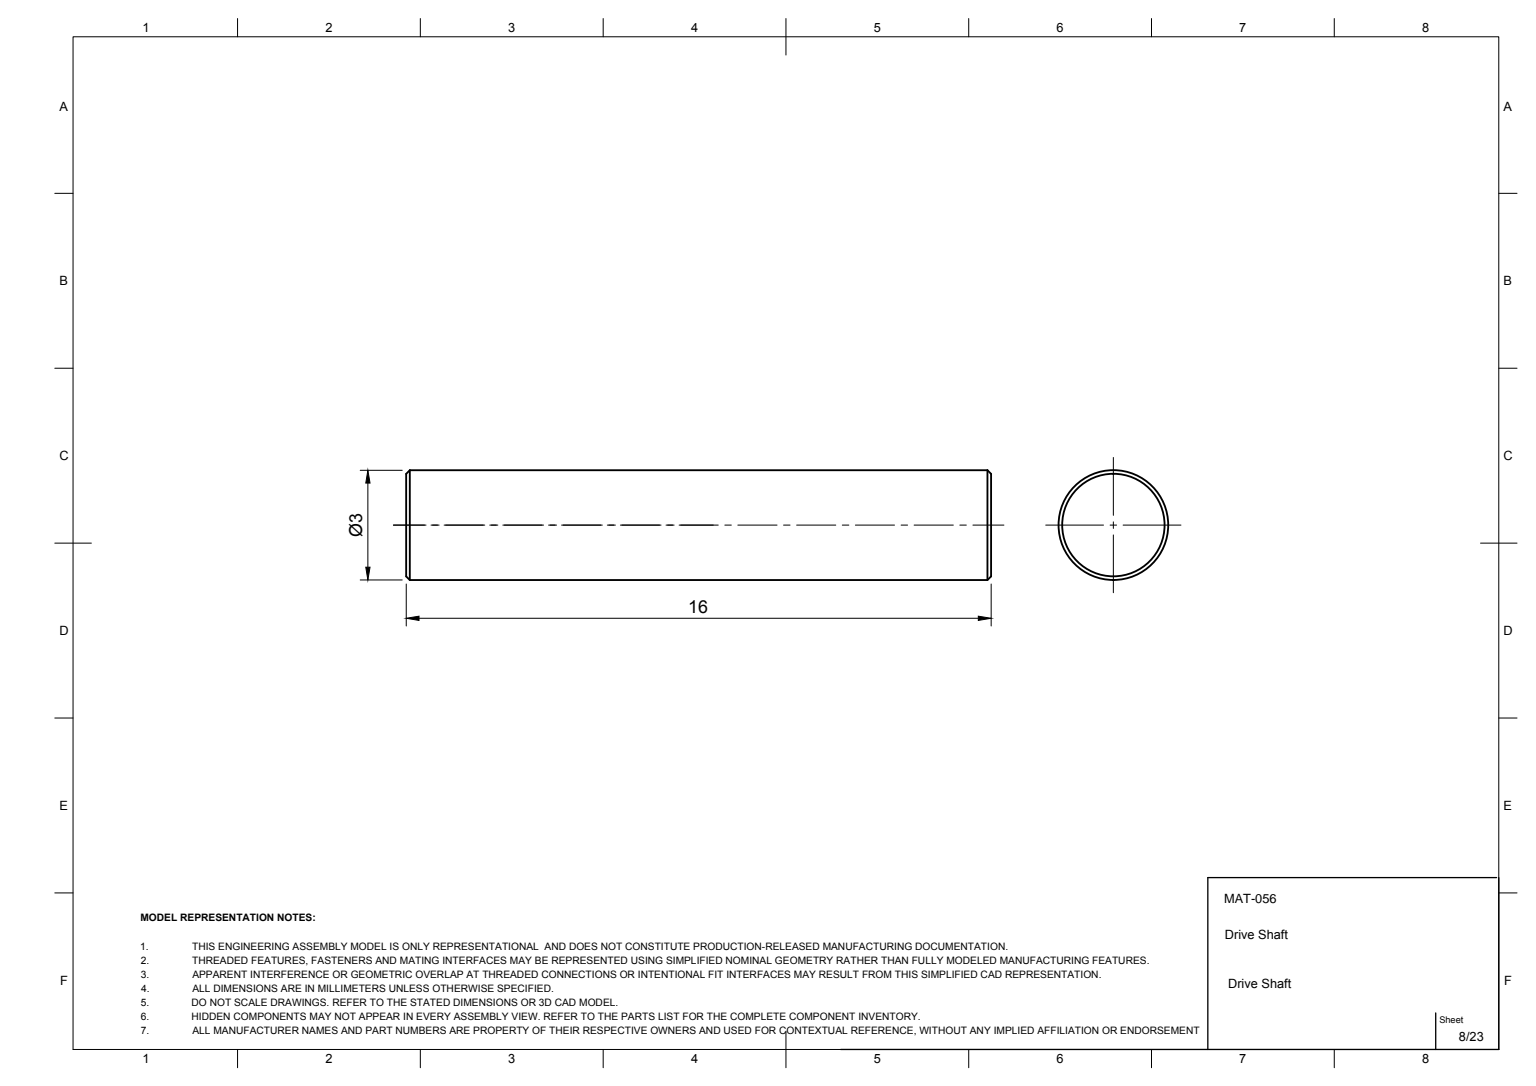
ISO-10303-21;
HEADER;
/* Generated by software containing ST-Developer
 * from STEP Tools, Inc. (www.steptools.com) 
 */

FILE_DESCRIPTION(
/* description */ (''),
/* implementation_level */ '2;1');

FILE_NAME(
/* name */ 'Drive Shaft.step',
/* time_stamp */ '2026-10-28T16:47:13+01:00',
/* author */ (''),
/* organization */ (''),
/* preprocessor_version */ 'ST-DEVELOPER v20.2',
/* originating_system */ 'Autodesk Translation Framework v15.17.0.0',
/* authorisation */ '');

FILE_SCHEMA (('AUTOMOTIVE_DESIGN { 1 0 10303 214 3 1 1 }'));
ENDSEC;

DATA;
#10=MECHANICAL_DESIGN_GEOMETRIC_PRESENTATION_REPRESENTATION('',(#4573),#459242);
#4410=SHAPE_REPRESENTATION_RELATIONSHIP('SRR','None',#459335,#4431);
#4431=ADVANCED_BREP_SHAPE_REPRESENTATION('',(#4453),#459224);
#4453=MANIFOLD_SOLID_BREP('Shaft body',#94631);
#4573=STYLED_ITEM('',(#459526),#4453);
#4710=CONICAL_SURFACE('',#97234,1.45,0.785398163397455);
#4711=CONICAL_SURFACE('',#97240,1.45,0.785398163397447);
#5589=PLANE('',#97239);
#5590=PLANE('',#97242);
#7435=FACE_OUTER_BOUND('',#13300,.T.);
#7436=FACE_OUTER_BOUND('',#13301,.T.);
#7437=FACE_OUTER_BOUND('',#13302,.T.);
#7438=FACE_OUTER_BOUND('',#13303,.T.);
#7439=FACE_OUTER_BOUND('',#13304,.T.);
#13300=EDGE_LOOP('',(#63820,#63821,#63822,#63823));
#13301=EDGE_LOOP('',(#63824,#63825,#63826,#63827));
#13302=EDGE_LOOP('',(#63828));
#13303=EDGE_LOOP('',(#63829,#63830,#63831,#63832));
#13304=EDGE_LOOP('',(#63833));
#19460=CIRCLE('',#97235,1.4);
#19461=CIRCLE('',#97236,1.5);
#19462=CIRCLE('',#97238,1.5);
#19463=CIRCLE('',#97241,1.4);
#28287=LINE('',#145861,#32089);
#28288=LINE('',#145866,#32090);
#28289=LINE('',#145871,#32091);
#32089=VECTOR('',#111479,1.45);
#32090=VECTOR('',#111486,1.5);
#32091=VECTOR('',#111493,1.45);
#36492=VERTEX_POINT('',#145858);
#36493=VERTEX_POINT('',#145860);
#36494=VERTEX_POINT('',#145864);
#36495=VERTEX_POINT('',#145869);
#46412=EDGE_CURVE('',#36492,#36492,#19460,.T.);
#46413=EDGE_CURVE('',#36492,#36493,#28287,.T.);
#46414=EDGE_CURVE('',#36493,#36493,#19461,.T.);
#46415=EDGE_CURVE('',#36494,#36494,#19462,.T.);
#46416=EDGE_CURVE('',#36494,#36493,#28288,.T.);
#46417=EDGE_CURVE('',#36495,#36495,#19463,.T.);
#46418=EDGE_CURVE('',#36495,#36494,#28289,.T.);
#63820=ORIENTED_EDGE('',*,*,#46412,.T.);
#63821=ORIENTED_EDGE('',*,*,#46413,.T.);
#63822=ORIENTED_EDGE('',*,*,#46414,.T.);
#63823=ORIENTED_EDGE('',*,*,#46413,.F.);
#63824=ORIENTED_EDGE('',*,*,#46415,.F.);
#63825=ORIENTED_EDGE('',*,*,#46416,.T.);
#63826=ORIENTED_EDGE('',*,*,#46414,.F.);
#63827=ORIENTED_EDGE('',*,*,#46416,.F.);
#63828=ORIENTED_EDGE('',*,*,#46412,.F.);
#63829=ORIENTED_EDGE('',*,*,#46417,.T.);
#63830=ORIENTED_EDGE('',*,*,#46418,.T.);
#63831=ORIENTED_EDGE('',*,*,#46415,.T.);
#63832=ORIENTED_EDGE('',*,*,#46418,.F.);
#63833=ORIENTED_EDGE('',*,*,#46417,.F.);
#87525=CYLINDRICAL_SURFACE('',#97237,1.5);
#89899=ADVANCED_FACE('',(#7435),#4710,.T.);
#89900=ADVANCED_FACE('',(#7436),#87525,.T.);
#89901=ADVANCED_FACE('',(#7437),#5589,.F.);
#89902=ADVANCED_FACE('',(#7438),#4711,.T.);
#89903=ADVANCED_FACE('',(#7439),#5590,.T.);
#94631=CLOSED_SHELL('',(#89899,#89900,#89901,#89902,#89903));
#97233=AXIS2_PLACEMENT_3D('',#145856,#111473,#111474);
#97234=AXIS2_PLACEMENT_3D('',#145857,#111475,#111476);
#97235=AXIS2_PLACEMENT_3D('',#145859,#111477,#111478);
#97236=AXIS2_PLACEMENT_3D('',#145862,#111480,#111481);
#97237=AXIS2_PLACEMENT_3D('',#145863,#111482,#111483);
#97238=AXIS2_PLACEMENT_3D('',#145865,#111484,#111485);
#97239=AXIS2_PLACEMENT_3D('',#145867,#111487,#111488);
#97240=AXIS2_PLACEMENT_3D('',#145868,#111489,#111490);
#97241=AXIS2_PLACEMENT_3D('',#145870,#111491,#111492);
#97242=AXIS2_PLACEMENT_3D('',#145872,#111494,#111495);
#111473=DIRECTION('axis',(0.,0.,1.));
#111474=DIRECTION('refdir',(1.,0.,0.));
#111475=DIRECTION('center_axis',(-3.56297039712382E-33,-1.,4.0245584642662E-16));
#111476=DIRECTION('ref_axis',(1.,-5.96129604355379E-16,3.46944695195422E-17));
#111477=DIRECTION('center_axis',(-5.55111512312578E-16,-1.,4.02455846426619E-16));
#111478=DIRECTION('ref_axis',(1.,-5.55111512312577E-16,3.46944695195422E-17));
#111479=DIRECTION('',(-0.707106781186552,-0.707106781186543,3.46642169093045E-16));
#111480=DIRECTION('center_axis',(5.55111512312578E-16,1.,-4.02455846426619E-16));
#111481=DIRECTION('ref_axis',(1.,-6.34413156928661E-16,3.46944695195423E-17));
#111482=DIRECTION('center_axis',(-6.34413156928661E-16,-1.,4.0245584642662E-16));
#111483=DIRECTION('ref_axis',(1.,-6.34413156928661E-16,3.46944695195423E-17));
#111484=DIRECTION('center_axis',(-5.55111512312578E-16,-1.,4.02455846426619E-16));
#111485=DIRECTION('ref_axis',(1.,-6.34413156928661E-16,3.46944695195423E-17));
#111486=DIRECTION('',(6.34413156928661E-16,1.,-4.0245584642662E-16));
#111487=DIRECTION('center_axis',(-5.55111512312578E-16,-1.,4.02455846426619E-16));
#111488=DIRECTION('ref_axis',(1.,-5.55111512312578E-16,3.46944695195422E-17));
#111489=DIRECTION('center_axis',(3.56297039712382E-33,1.,-4.0245584642662E-16));
#111490=DIRECTION('ref_axis',(1.,-5.96129604355379E-16,3.46944695195422E-17));
#111491=DIRECTION('center_axis',(5.55111512312578E-16,1.,-4.02455846426619E-16));
#111492=DIRECTION('ref_axis',(1.,-5.55111512312578E-16,3.46944695195422E-17));
#111493=DIRECTION('',(-0.707106781186547,0.707106781186548,-3.95707558426922E-16));
#111494=DIRECTION('center_axis',(-5.55111512312578E-16,-1.,4.02455846426619E-16));
#111495=DIRECTION('ref_axis',(1.,-5.55111512312578E-16,3.46944695195422E-17));
#145856=CARTESIAN_POINT('',(0.,0.,0.));
#145857=CARTESIAN_POINT('Origin',(-8.84687992363536,110.965520572543,16.0678367667527));
#145858=CARTESIAN_POINT('',(-10.2468799236354,111.015520572543,16.0678367667527));
#145859=CARTESIAN_POINT('Origin',(-8.84687992363536,111.015520572543,16.0678367667527));
#145860=CARTESIAN_POINT('',(-10.3468799236354,110.915520572543,16.0678367667527));
#145861=CARTESIAN_POINT('',(-10.2968799236354,110.965520572543,16.0678367667527));
#145862=CARTESIAN_POINT('Origin',(-8.84687992363536,110.915520572543,16.0678367667527));
#145863=CARTESIAN_POINT('Origin',(-8.84687992363537,98.5155205725429,16.0678367667527));
#145864=CARTESIAN_POINT('',(-10.3468799236354,95.1155205725429,16.0678367667528));
#145865=CARTESIAN_POINT('Origin',(-8.84687992363537,95.1155205725429,16.0678367667528));
#145866=CARTESIAN_POINT('',(-10.3468799236354,98.5155205725429,16.0678367667527));
#145867=CARTESIAN_POINT('Origin',(-8.84687992363536,111.015520572543,16.0678367667527));
#145868=CARTESIAN_POINT('Origin',(-8.84687992363537,95.065520572543,16.0678367667528));
#145869=CARTESIAN_POINT('',(-10.2468799236354,95.0155205725429,16.0678367667528));
#145870=CARTESIAN_POINT('Origin',(-8.84687992363537,95.0155205725429,16.0678367667528));
#145871=CARTESIAN_POINT('',(-10.2968799236354,95.065520572543,16.0678367667528));
#145872=CARTESIAN_POINT('Origin',(-8.84687992363537,95.0155205725429,16.0678367667528));
#459198=UNCERTAINTY_MEASURE_WITH_UNIT(LENGTH_MEASURE(0.01),#459243,
'DISTANCE_ACCURACY_VALUE',
'Maximum model space distance between geometric entities at asserted c
onnectivities');
#459216=UNCERTAINTY_MEASURE_WITH_UNIT(LENGTH_MEASURE(0.01),#459243,
'DISTANCE_ACCURACY_VALUE',
'Maximum model space distance between geometric entities at asserted c
onnectivities');
#459224=(
GEOMETRIC_REPRESENTATION_CONTEXT(3)
GLOBAL_UNCERTAINTY_ASSIGNED_CONTEXT((#459198))
GLOBAL_UNIT_ASSIGNED_CONTEXT((#459243,#459245,#459246))
REPRESENTATION_CONTEXT('','3D')
);
#459242=(
GEOMETRIC_REPRESENTATION_CONTEXT(3)
GLOBAL_UNCERTAINTY_ASSIGNED_CONTEXT((#459216))
GLOBAL_UNIT_ASSIGNED_CONTEXT((#459243,#459245,#459246))
REPRESENTATION_CONTEXT('','3D')
);
#459243=(
LENGTH_UNIT()
NAMED_UNIT(*)
SI_UNIT(.MILLI.,.METRE.)
);
#459245=(
NAMED_UNIT(*)
PLANE_ANGLE_UNIT()
SI_UNIT($,.RADIAN.)
);
#459246=(
NAMED_UNIT(*)
SI_UNIT($,.STERADIAN.)
SOLID_ANGLE_UNIT()
);
#459254=SHAPE_DEFINITION_REPRESENTATION(#459279,#459335);
#459279=PRODUCT_DEFINITION_SHAPE('',$,#459361);
#459335=SHAPE_REPRESENTATION('',(#97233),#459224);
#459353=PRODUCT_DEFINITION_CONTEXT('part definition',#459430,'design');
#459361=PRODUCT_DEFINITION('Drive Shaft','Drive Shaft',#459386,#459353);
#459386=PRODUCT_DEFINITION_FORMATION('',$,#459439);
#459430=APPLICATION_CONTEXT(
'Core Data for Automotive Mechanical Design Process');
#459431=PRODUCT_CONTEXT('part definition',#459430,'mechanical');
#459439=PRODUCT('Drive Shaft','Drive Shaft',$,(#459431));
#459520=COLOUR_RGB('Grey',0.48,0.52,0.57);
#459521=FILL_AREA_STYLE_COLOUR('',#459520);
#459522=FILL_AREA_STYLE('',(#459521));
#459523=SURFACE_STYLE_FILL_AREA(#459522);
#459524=SURFACE_SIDE_STYLE('',(#459523));
#459525=SURFACE_STYLE_USAGE(.BOTH.,#459524);
#459526=PRESENTATION_STYLE_ASSIGNMENT((#459525));
ENDSEC;
END-ISO-10303-21;
